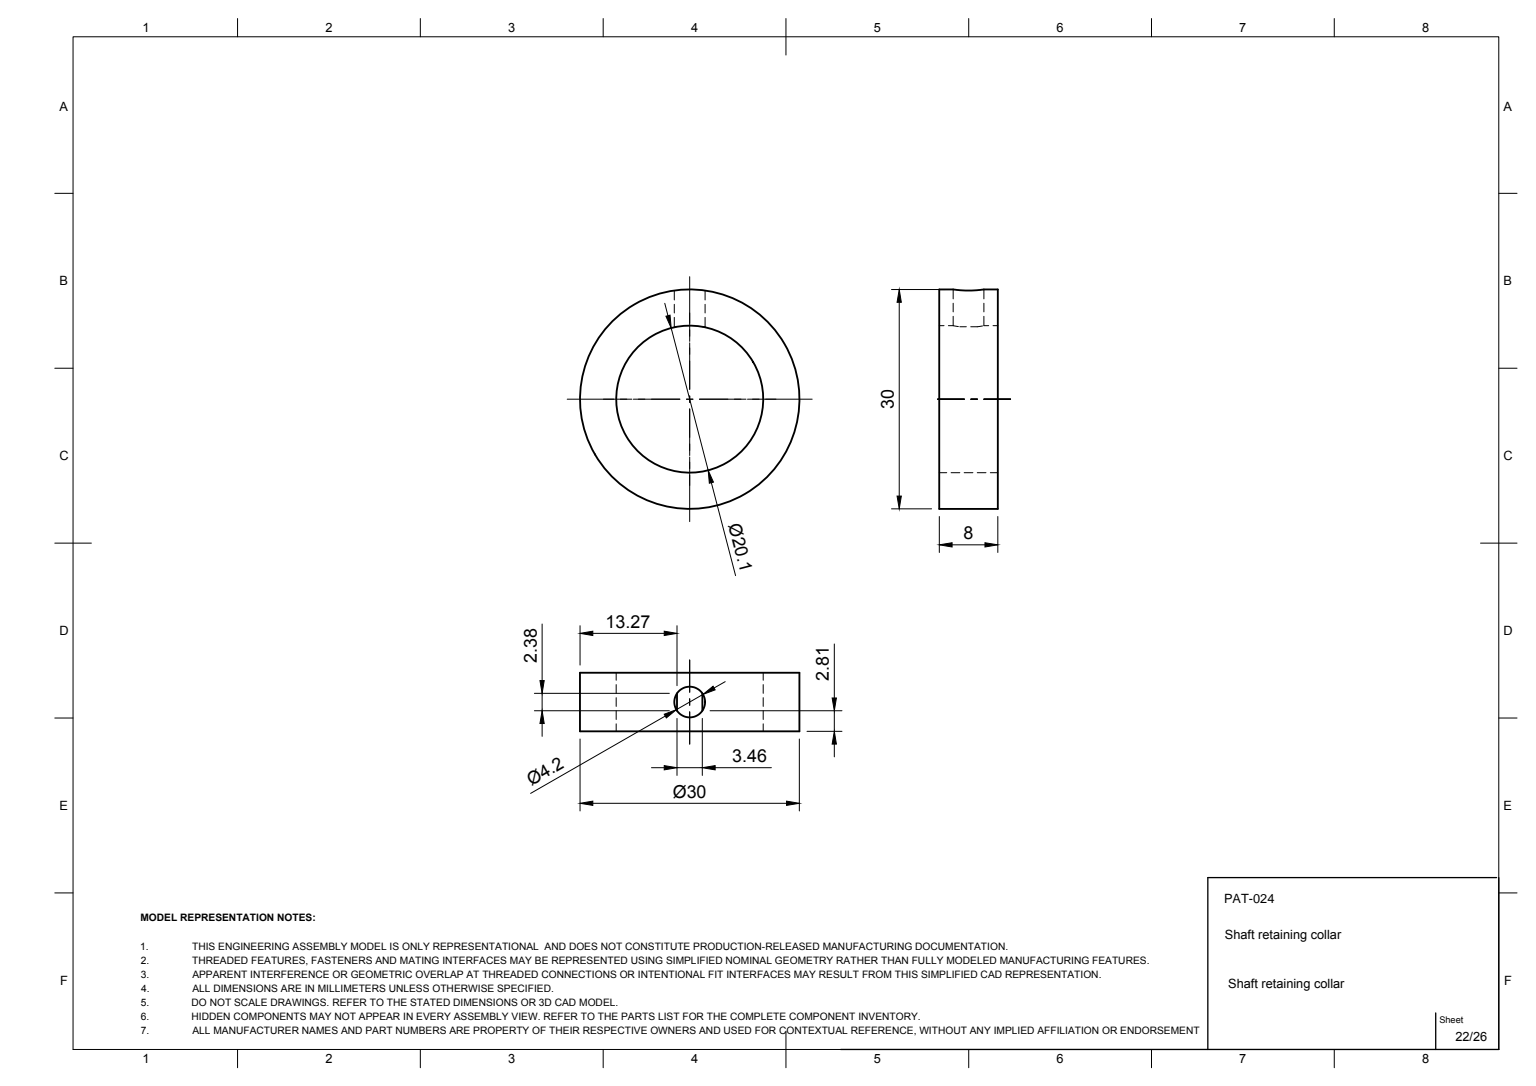
ISO-10303-21;
HEADER;
/* Generated by software containing ST-Developer
 * from STEP Tools, Inc. (www.steptools.com) 
 */

FILE_DESCRIPTION(
/* description */ ('Compact handwheel screw vise'),
/* implementation_level */ '2;1');

FILE_NAME(
/* name */ 'Shaft retaining collar.step',
/* time_stamp */ '2026-10-29T16:08:22-07:00',
/* author */ (''),
/* organization */ (''),
/* preprocessor_version */ 'ST-DEVELOPER v20.2',
/* originating_system */ 'Autodesk Translation Framework v15.17.0.0',
/* authorisation */ '');

FILE_SCHEMA (('AUTOMOTIVE_DESIGN { 1 0 10303 214 3 1 1 }'));
ENDSEC;

DATA;
#10=MECHANICAL_DESIGN_GEOMETRIC_PRESENTATION_REPRESENTATION('',(#672),#25074);
#531=B_SPLINE_CURVE_WITH_KNOTS('',3,(#24543,#24544,#24545,#24546,#24547,
#24548,#24549,#24550),.UNSPECIFIED.,.F.,.F.,(4,2,2,4),(0.756005737987019,
0.793568827564653,0.872922520054208,0.952276212543762),.UNSPECIFIED.);
#532=B_SPLINE_CURVE_WITH_KNOTS('',3,(#24553,#24554,#24555,#24556,#24557,
#24558,#24559,#24560,#24561,#24562,#24563,#24564,#24565,#24566),
 .UNSPECIFIED.,.F.,.F.,(4,2,2,2,2,2,4),(0.121154929624509,0.158718019202145,
0.238071711691699,0.317425404181254,0.396779096670809,0.476132789160363,
0.513695878738001),.UNSPECIFIED.);
#533=B_SPLINE_CURVE_WITH_KNOTS('',3,(#24567,#24568,#24569,#24570,#24571,
#24572,#24573,#24574),.UNSPECIFIED.,.F.,.F.,(4,2,2,4),(0.952276212543762,
1.03162990503332,1.11098359752287,1.14854668710052),.UNSPECIFIED.);
#534=B_SPLINE_CURVE_WITH_KNOTS('',3,(#24578,#24579,#24580,#24581,#24582,
#24583,#24584,#24585,#24586,#24587),.UNSPECIFIED.,.F.,.F.,(4,2,2,2,4),(0.,
0.0792165807733642,0.158433161546728,0.237648697074572,0.316864232602417),
 .UNSPECIFIED.);
#535=B_SPLINE_CURVE_WITH_KNOTS('',3,(#24588,#24589,#24590,#24591,#24592,
#24593,#24594,#24595,#24596,#24597,#24598,#24599,#24600,#24601,#24602,#24603,
#24604,#24605,#24606,#24607,#24608,#24609,#24610,#24611,#24612,#24613),
 .UNSPECIFIED.,.F.,.F.,(4,2,2,2,2,2,2,2,2,2,2,2,4),(0.316864232602417,0.396079768130261,
0.475295303658105,0.554511884431469,0.633728465204833,0.712945045978197,
0.792161626751562,0.871377162279406,0.95059269780725,1.02980823333509,1.10902376886294,
1.1882403496363,1.26745693040967),.UNSPECIFIED.);
#608=SHAPE_REPRESENTATION_RELATIONSHIP('SRR','None',#25219,#636);
#636=ADVANCED_BREP_SHAPE_REPRESENTATION('',(#705),#25066);
#672=STYLED_ITEM('',(#25439),#705);
#705=MANIFOLD_SOLID_BREP('Body1',#8083);
#804=FACE_BOUND('',#1977,.T.);
#805=FACE_BOUND('',#1979,.T.);
#806=FACE_BOUND('',#1981,.T.);
#807=FACE_BOUND('',#1983,.T.);
#964=PLANE('',#9053);
#965=PLANE('',#9057);
#966=PLANE('',#9064);
#967=PLANE('',#9065);
#1411=FACE_OUTER_BOUND('',#1973,.T.);
#1412=FACE_OUTER_BOUND('',#1974,.T.);
#1413=FACE_OUTER_BOUND('',#1975,.T.);
#1414=FACE_OUTER_BOUND('',#1976,.T.);
#1415=FACE_OUTER_BOUND('',#1978,.T.);
#1416=FACE_OUTER_BOUND('',#1980,.T.);
#1417=FACE_OUTER_BOUND('',#1982,.T.);
#1973=EDGE_LOOP('',(#7047,#7048));
#1974=EDGE_LOOP('',(#7049,#7050,#7051,#7052,#7053,#7054,#7055,#7056,#7057));
#1975=EDGE_LOOP('',(#7058,#7059));
#1976=EDGE_LOOP('',(#7060,#7061,#7062,#7063));
#1977=EDGE_LOOP('',(#7064,#7065,#7066,#7067,#7068));
#1978=EDGE_LOOP('',(#7069,#7070,#7071,#7072));
#1979=EDGE_LOOP('',(#7073,#7074));
#1980=EDGE_LOOP('',(#7075));
#1981=EDGE_LOOP('',(#7076));
#1982=EDGE_LOOP('',(#7077));
#1983=EDGE_LOOP('',(#7078));
#2471=LINE('',#24538,#2979);
#2472=LINE('',#24576,#2980);
#2473=LINE('',#24615,#2981);
#2474=LINE('',#24620,#2982);
#2475=LINE('',#24626,#2983);
#2979=VECTOR('',#10919,1.);
#2980=VECTOR('',#10926,0.210000000000001);
#2981=VECTOR('',#10929,1.);
#2982=VECTOR('',#10934,1.005);
#2983=VECTOR('',#10941,1.5);
#3293=CIRCLE('',#9054,0.210000000000001);
#3294=CIRCLE('',#9056,0.210000000000001);
#3295=CIRCLE('',#9059,1.005);
#3296=CIRCLE('',#9060,1.005);
#3297=CIRCLE('',#9062,1.5);
#3298=CIRCLE('',#9063,1.5);
#3968=VERTEX_POINT('',#24536);
#3969=VERTEX_POINT('',#24537);
#3970=VERTEX_POINT('',#24541);
#3971=VERTEX_POINT('',#24542);
#3972=VERTEX_POINT('',#24551);
#3973=VERTEX_POINT('',#24575);
#3974=VERTEX_POINT('',#24577);
#3975=VERTEX_POINT('',#24617);
#3976=VERTEX_POINT('',#24619);
#3977=VERTEX_POINT('',#24623);
#3978=VERTEX_POINT('',#24625);
#5010=EDGE_CURVE('',#3968,#3969,#2471,.T.);
#5011=EDGE_CURVE('',#3968,#3969,#3293,.T.);
#5012=EDGE_CURVE('',#3970,#3971,#531,.T.);
#5013=EDGE_CURVE('',#3972,#3970,#3294,.T.);
#5014=EDGE_CURVE('',#3969,#3972,#532,.T.);
#5015=EDGE_CURVE('',#3971,#3968,#533,.T.);
#5016=EDGE_CURVE('',#3971,#3973,#2472,.T.);
#5017=EDGE_CURVE('',#3974,#3973,#534,.T.);
#5018=EDGE_CURVE('',#3973,#3974,#535,.T.);
#5019=EDGE_CURVE('',#3972,#3970,#2473,.T.);
#5020=EDGE_CURVE('',#3975,#3975,#3295,.T.);
#5021=EDGE_CURVE('',#3975,#3976,#2474,.T.);
#5022=EDGE_CURVE('',#3976,#3976,#3296,.T.);
#5023=EDGE_CURVE('',#3977,#3977,#3297,.T.);
#5024=EDGE_CURVE('',#3977,#3978,#2475,.T.);
#5025=EDGE_CURVE('',#3978,#3978,#3298,.T.);
#7047=ORIENTED_EDGE('',*,*,#5010,.F.);
#7048=ORIENTED_EDGE('',*,*,#5011,.T.);
#7049=ORIENTED_EDGE('',*,*,#5012,.F.);
#7050=ORIENTED_EDGE('',*,*,#5013,.F.);
#7051=ORIENTED_EDGE('',*,*,#5014,.F.);
#7052=ORIENTED_EDGE('',*,*,#5011,.F.);
#7053=ORIENTED_EDGE('',*,*,#5015,.F.);
#7054=ORIENTED_EDGE('',*,*,#5016,.T.);
#7055=ORIENTED_EDGE('',*,*,#5017,.F.);
#7056=ORIENTED_EDGE('',*,*,#5018,.F.);
#7057=ORIENTED_EDGE('',*,*,#5016,.F.);
#7058=ORIENTED_EDGE('',*,*,#5019,.F.);
#7059=ORIENTED_EDGE('',*,*,#5013,.T.);
#7060=ORIENTED_EDGE('',*,*,#5020,.F.);
#7061=ORIENTED_EDGE('',*,*,#5021,.T.);
#7062=ORIENTED_EDGE('',*,*,#5022,.T.);
#7063=ORIENTED_EDGE('',*,*,#5021,.F.);
#7064=ORIENTED_EDGE('',*,*,#5014,.T.);
#7065=ORIENTED_EDGE('',*,*,#5019,.T.);
#7066=ORIENTED_EDGE('',*,*,#5012,.T.);
#7067=ORIENTED_EDGE('',*,*,#5015,.T.);
#7068=ORIENTED_EDGE('',*,*,#5010,.T.);
#7069=ORIENTED_EDGE('',*,*,#5023,.F.);
#7070=ORIENTED_EDGE('',*,*,#5024,.T.);
#7071=ORIENTED_EDGE('',*,*,#5025,.T.);
#7072=ORIENTED_EDGE('',*,*,#5024,.F.);
#7073=ORIENTED_EDGE('',*,*,#5017,.T.);
#7074=ORIENTED_EDGE('',*,*,#5018,.T.);
#7075=ORIENTED_EDGE('',*,*,#5023,.T.);
#7076=ORIENTED_EDGE('',*,*,#5020,.T.);
#7077=ORIENTED_EDGE('',*,*,#5025,.F.);
#7078=ORIENTED_EDGE('',*,*,#5022,.F.);
#7565=CYLINDRICAL_SURFACE('',#9055,0.210000000000001);
#7566=CYLINDRICAL_SURFACE('',#9058,1.005);
#7567=CYLINDRICAL_SURFACE('',#9061,1.5);
#7981=ADVANCED_FACE('',(#1411),#964,.T.);
#7982=ADVANCED_FACE('',(#1412),#7565,.F.);
#7983=ADVANCED_FACE('',(#1413),#965,.T.);
#7984=ADVANCED_FACE('',(#1414,#804),#7566,.F.);
#7985=ADVANCED_FACE('',(#1415,#805),#7567,.T.);
#7986=ADVANCED_FACE('',(#1416,#806),#966,.T.);
#7987=ADVANCED_FACE('',(#1417,#807),#967,.F.);
#8083=CLOSED_SHELL('',(#7981,#7982,#7983,#7984,#7985,#7986,#7987));
#9052=AXIS2_PLACEMENT_3D('',#24534,#10915,#10916);
#9053=AXIS2_PLACEMENT_3D('',#24535,#10917,#10918);
#9054=AXIS2_PLACEMENT_3D('',#24539,#10920,#10921);
#9055=AXIS2_PLACEMENT_3D('',#24540,#10922,#10923);
#9056=AXIS2_PLACEMENT_3D('',#24552,#10924,#10925);
#9057=AXIS2_PLACEMENT_3D('',#24614,#10927,#10928);
#9058=AXIS2_PLACEMENT_3D('',#24616,#10930,#10931);
#9059=AXIS2_PLACEMENT_3D('',#24618,#10932,#10933);
#9060=AXIS2_PLACEMENT_3D('',#24621,#10935,#10936);
#9061=AXIS2_PLACEMENT_3D('',#24622,#10937,#10938);
#9062=AXIS2_PLACEMENT_3D('',#24624,#10939,#10940);
#9063=AXIS2_PLACEMENT_3D('',#24627,#10942,#10943);
#9064=AXIS2_PLACEMENT_3D('',#24628,#10944,#10945);
#9065=AXIS2_PLACEMENT_3D('',#24629,#10946,#10947);
#10915=DIRECTION('axis',(0.,0.,1.));
#10916=DIRECTION('refdir',(1.,0.,0.));
#10917=DIRECTION('center_axis',(0.,1.,0.));
#10918=DIRECTION('ref_axis',(1.,0.,0.));
#10919=DIRECTION('',(1.,0.,0.));
#10920=DIRECTION('center_axis',(0.,1.,0.));
#10921=DIRECTION('ref_axis',(1.,0.,0.));
#10922=DIRECTION('center_axis',(0.,1.,0.));
#10923=DIRECTION('ref_axis',(1.,0.,0.));
#10924=DIRECTION('center_axis',(0.,1.,0.));
#10925=DIRECTION('ref_axis',(1.,0.,0.));
#10926=DIRECTION('',(0.,1.,0.));
#10927=DIRECTION('center_axis',(0.,1.,0.));
#10928=DIRECTION('ref_axis',(1.,0.,0.));
#10929=DIRECTION('',(-1.,0.,0.));
#10930=DIRECTION('center_axis',(1.,0.,0.));
#10931=DIRECTION('ref_axis',(0.,0.,-1.));
#10932=DIRECTION('center_axis',(-1.,0.,0.));
#10933=DIRECTION('ref_axis',(0.,0.,-1.));
#10934=DIRECTION('',(-1.,0.,0.));
#10935=DIRECTION('center_axis',(-1.,0.,0.));
#10936=DIRECTION('ref_axis',(0.,0.,-1.));
#10937=DIRECTION('center_axis',(1.,0.,0.));
#10938=DIRECTION('ref_axis',(0.,0.,-1.));
#10939=DIRECTION('center_axis',(1.,0.,0.));
#10940=DIRECTION('ref_axis',(0.,0.,-1.));
#10941=DIRECTION('',(-1.,0.,0.));
#10942=DIRECTION('center_axis',(1.,0.,0.));
#10943=DIRECTION('ref_axis',(0.,0.,-1.));
#10944=DIRECTION('center_axis',(1.,0.,0.));
#10945=DIRECTION('ref_axis',(0.,0.,-1.));
#10946=DIRECTION('center_axis',(1.,0.,0.));
#10947=DIRECTION('ref_axis',(0.,0.,-1.));
#24534=CARTESIAN_POINT('',(0.,0.,0.));
#24535=CARTESIAN_POINT('Origin',(25.8,0.99,4.));
#24536=CARTESIAN_POINT('',(25.6809411910021,0.99,4.17298843892006));
#24537=CARTESIAN_POINT('',(25.9190588089979,0.99,4.17298843892006));
#24538=CARTESIAN_POINT('',(25.4,0.99,4.17298843892006));
#24539=CARTESIAN_POINT('Origin',(25.8,0.99,4.));
#24540=CARTESIAN_POINT('Origin',(25.8,0.99,4.));
#24541=CARTESIAN_POINT('',(25.6809411910021,0.99,3.82701156107994));
#24542=CARTESIAN_POINT('',(25.59,1.005,4.));
#24543=CARTESIAN_POINT('Ctrl Pts',(25.6809411910021,0.989999999999999,3.82701156107994));
#24544=CARTESIAN_POINT('Ctrl Pts',(25.6701985776047,0.99129192197638,3.83440513468868));
#24545=CARTESIAN_POINT('Ctrl Pts',(25.6603122906273,0.992653949439047,3.84270286127439));
#24546=CARTESIAN_POINT('Ctrl Pts',(25.6329072257467,0.996748084390898,3.87010792615492));
#24547=CARTESIAN_POINT('Ctrl Pts',(25.6167579436671,0.999695893276376,3.89366983224072));
#24548=CARTESIAN_POINT('Ctrl Pts',(25.5953022060351,1.00385029472357,3.94538709536759));
#24549=CARTESIAN_POINT('Ctrl Pts',(25.59,1.005,3.97354876917015));
#24550=CARTESIAN_POINT('Ctrl Pts',(25.59,1.005,4.));
#24551=CARTESIAN_POINT('',(25.9190588089979,0.99,3.82701156107994));
#24552=CARTESIAN_POINT('Origin',(25.8,0.99,4.));
#24553=CARTESIAN_POINT('Ctrl Pts',(25.9190588089979,0.99,4.17298843892006));
#24554=CARTESIAN_POINT('Ctrl Pts',(25.9298014223953,0.991291921976381,4.16559486531132));
#24555=CARTESIAN_POINT('Ctrl Pts',(25.9396877093727,0.992653949439047,4.15729713872561));
#24556=CARTESIAN_POINT('Ctrl Pts',(25.9670927742533,0.996748084390898,4.12989207384508));
#24557=CARTESIAN_POINT('Ctrl Pts',(25.9832420563329,0.999695893276376,4.10633016775929));
#24558=CARTESIAN_POINT('Ctrl Pts',(26.0046977939649,1.00385029472357,4.05461290463241));
#24559=CARTESIAN_POINT('Ctrl Pts',(26.01,1.005,4.02645123082985));
#24560=CARTESIAN_POINT('Ctrl Pts',(26.01,1.005,3.97354876917015));
#24561=CARTESIAN_POINT('Ctrl Pts',(26.0046977939649,1.00385029472357,3.94538709536759));
#24562=CARTESIAN_POINT('Ctrl Pts',(25.9832420563329,0.999695893276376,3.89366983224072));
#24563=CARTESIAN_POINT('Ctrl Pts',(25.9670927742533,0.996748084390898,3.87010792615492));
#24564=CARTESIAN_POINT('Ctrl Pts',(25.9396877093727,0.992653949439047,3.84270286127439));
#24565=CARTESIAN_POINT('Ctrl Pts',(25.9298014223953,0.991291921976381,3.83440513468868));
#24566=CARTESIAN_POINT('Ctrl Pts',(25.9190588089979,0.99,3.82701156107994));
#24567=CARTESIAN_POINT('Ctrl Pts',(25.59,1.005,4.));
#24568=CARTESIAN_POINT('Ctrl Pts',(25.59,1.005,4.02645123082985));
#24569=CARTESIAN_POINT('Ctrl Pts',(25.5953022060351,1.00385029472357,4.05461290463241));
#24570=CARTESIAN_POINT('Ctrl Pts',(25.6167579436671,0.999695893276376,4.10633016775929));
#24571=CARTESIAN_POINT('Ctrl Pts',(25.6329072257467,0.996748084390898,4.12989207384508));
#24572=CARTESIAN_POINT('Ctrl Pts',(25.6603122906273,0.992653949439047,4.15729713872561));
#24573=CARTESIAN_POINT('Ctrl Pts',(25.6701985776047,0.991291921976381,4.16559486531132));
#24574=CARTESIAN_POINT('Ctrl Pts',(25.6809411910021,0.99,4.17298843892006));
#24575=CARTESIAN_POINT('',(25.59,1.5,4.));
#24576=CARTESIAN_POINT('',(25.59,0.99,4.));
#24577=CARTESIAN_POINT('',(25.8,1.48522725533839,4.21));
#24578=CARTESIAN_POINT('Ctrl Pts',(25.8,1.48522725533839,4.21));
#24579=CARTESIAN_POINT('Ctrl Pts',(25.7735944730755,1.48522725533839,4.21));
#24580=CARTESIAN_POINT('Ctrl Pts',(25.7454529259093,1.48600415954412,4.2047157372696));
#24581=CARTESIAN_POINT('Ctrl Pts',(25.6937237310949,1.48880073282317,4.18327376303633));
#24582=CARTESIAN_POINT('Ctrl Pts',(25.670133075872,1.49077897157582,4.16711792397039));
#24583=CARTESIAN_POINT('Ctrl Pts',(25.632882321789,1.49448481141327,4.12986716988737));
#24584=CARTESIAN_POINT('Ctrl Pts',(25.6167262899986,1.49645455657129,4.10627640830577));
#24585=CARTESIAN_POINT('Ctrl Pts',(25.5952841751738,1.49923165515646,4.0545468514059));
#24586=CARTESIAN_POINT('Ctrl Pts',(25.59,1.5,4.02640517850928));
#24587=CARTESIAN_POINT('Ctrl Pts',(25.59,1.5,4.));
#24588=CARTESIAN_POINT('Ctrl Pts',(25.59,1.5,4.));
#24589=CARTESIAN_POINT('Ctrl Pts',(25.59,1.5,3.97359482149072));
#24590=CARTESIAN_POINT('Ctrl Pts',(25.5952841751738,1.49923165515646,3.9454531485941));
#24591=CARTESIAN_POINT('Ctrl Pts',(25.6167262899986,1.49645455657129,3.89372359169423));
#24592=CARTESIAN_POINT('Ctrl Pts',(25.632882321789,1.49448481141327,3.87013283011263));
#24593=CARTESIAN_POINT('Ctrl Pts',(25.670133075872,1.49077897157582,3.83288207602961));
#24594=CARTESIAN_POINT('Ctrl Pts',(25.6937237310949,1.48880073282317,3.81672623696366));
#24595=CARTESIAN_POINT('Ctrl Pts',(25.7454529259093,1.48600415954412,3.7952842627304));
#24596=CARTESIAN_POINT('Ctrl Pts',(25.7735944730755,1.48522725533839,3.79));
#24597=CARTESIAN_POINT('Ctrl Pts',(25.8264055269245,1.48522725533839,3.79));
#24598=CARTESIAN_POINT('Ctrl Pts',(25.8545470740907,1.48600415954412,3.7952842627304));
#24599=CARTESIAN_POINT('Ctrl Pts',(25.9062762689051,1.48880073282317,3.81672623696367));
#24600=CARTESIAN_POINT('Ctrl Pts',(25.929866924128,1.49077897157582,3.83288207602961));
#24601=CARTESIAN_POINT('Ctrl Pts',(25.967117678211,1.49448481141327,3.87013283011263));
#24602=CARTESIAN_POINT('Ctrl Pts',(25.9832737100014,1.49645455657129,3.89372359169423));
#24603=CARTESIAN_POINT('Ctrl Pts',(26.0047158248262,1.49923165515646,3.9454531485941));
#24604=CARTESIAN_POINT('Ctrl Pts',(26.01,1.5,3.97359482149072));
#24605=CARTESIAN_POINT('Ctrl Pts',(26.01,1.5,4.02640517850928));
#24606=CARTESIAN_POINT('Ctrl Pts',(26.0047158248262,1.49923165515646,4.0545468514059));
#24607=CARTESIAN_POINT('Ctrl Pts',(25.9832737100014,1.49645455657129,4.10627640830577));
#24608=CARTESIAN_POINT('Ctrl Pts',(25.967117678211,1.49448481141327,4.12986716988737));
#24609=CARTESIAN_POINT('Ctrl Pts',(25.929866924128,1.49077897157582,4.16711792397039));
#24610=CARTESIAN_POINT('Ctrl Pts',(25.9062762689051,1.48880073282317,4.18327376303633));
#24611=CARTESIAN_POINT('Ctrl Pts',(25.8545470740907,1.48600415954412,4.20471573726959));
#24612=CARTESIAN_POINT('Ctrl Pts',(25.8264055269245,1.48522725533839,4.21));
#24613=CARTESIAN_POINT('Ctrl Pts',(25.8,1.48522725533839,4.21));
#24614=CARTESIAN_POINT('Origin',(25.8,0.99,4.));
#24615=CARTESIAN_POINT('',(25.4,0.99,3.82701156107994));
#24616=CARTESIAN_POINT('Origin',(25.4,0.,4.));
#24617=CARTESIAN_POINT('',(26.2,-1.23077003314309E-16,5.005));
#24618=CARTESIAN_POINT('Origin',(26.2,0.,4.));
#24619=CARTESIAN_POINT('',(25.4,-1.23077003314309E-16,5.005));
#24620=CARTESIAN_POINT('',(25.4,-1.23077003314309E-16,5.005));
#24621=CARTESIAN_POINT('Origin',(25.4,0.,4.));
#24622=CARTESIAN_POINT('Origin',(25.4,0.,4.));
#24623=CARTESIAN_POINT('',(26.2,-1.83697019872103E-16,5.5));
#24624=CARTESIAN_POINT('Origin',(26.2,0.,4.));
#24625=CARTESIAN_POINT('',(25.4,-1.83697019872103E-16,5.5));
#24626=CARTESIAN_POINT('',(25.4,-1.83697019872103E-16,5.5));
#24627=CARTESIAN_POINT('Origin',(25.4,0.,4.));
#24628=CARTESIAN_POINT('Origin',(26.2,0.,4.));
#24629=CARTESIAN_POINT('Origin',(25.4,0.,4.));
#25032=UNCERTAINTY_MEASURE_WITH_UNIT(LENGTH_MEASURE(0.001),#25075,
'DISTANCE_ACCURACY_VALUE',
'Maximum model space distance between geometric entities at asserted c
onnectivities');
#25040=UNCERTAINTY_MEASURE_WITH_UNIT(LENGTH_MEASURE(0.001),#25075,
'DISTANCE_ACCURACY_VALUE',
'Maximum model space distance between geometric entities at asserted c
onnectivities');
#25066=(
GEOMETRIC_REPRESENTATION_CONTEXT(3)
GLOBAL_UNCERTAINTY_ASSIGNED_CONTEXT((#25032))
GLOBAL_UNIT_ASSIGNED_CONTEXT((#25075,#25077,#25078))
REPRESENTATION_CONTEXT('','3D')
);
#25074=(
GEOMETRIC_REPRESENTATION_CONTEXT(3)
GLOBAL_UNCERTAINTY_ASSIGNED_CONTEXT((#25040))
GLOBAL_UNIT_ASSIGNED_CONTEXT((#25075,#25077,#25078))
REPRESENTATION_CONTEXT('','3D')
);
#25075=(
LENGTH_UNIT()
NAMED_UNIT(*)
SI_UNIT(.CENTI.,.METRE.)
);
#25077=(
NAMED_UNIT(*)
PLANE_ANGLE_UNIT()
SI_UNIT($,.RADIAN.)
);
#25078=(
NAMED_UNIT(*)
SI_UNIT($,.STERADIAN.)
SOLID_ANGLE_UNIT()
);
#25104=SHAPE_DEFINITION_REPRESENTATION(#25153,#25219);
#25153=PRODUCT_DEFINITION_SHAPE('',$,#25253);
#25219=SHAPE_REPRESENTATION('',(#9052),#25066);
#25227=PRODUCT_DEFINITION_CONTEXT('part definition',#25328,'design');
#25253=PRODUCT_DEFINITION('Shaft retaining collar',
'Shaft retaining collar',#25286,#25227);
#25286=PRODUCT_DEFINITION_FORMATION('',$,#25355);
#25328=APPLICATION_CONTEXT(
'Core Data for Automotive Mechanical Design Process');
#25329=PRODUCT_CONTEXT('part definition',#25328,'mechanical');
#25355=PRODUCT('Shaft retaining collar','Shaft retaining collar',
'Shaft retaining collar',(#25329));
#25433=COLOUR_RGB('Grey',0.48,0.52,0.57);
#25434=FILL_AREA_STYLE_COLOUR('',#25433);
#25435=FILL_AREA_STYLE('',(#25434));
#25436=SURFACE_STYLE_FILL_AREA(#25435);
#25437=SURFACE_SIDE_STYLE('',(#25436));
#25438=SURFACE_STYLE_USAGE(.BOTH.,#25437);
#25439=PRESENTATION_STYLE_ASSIGNMENT((#25438));
ENDSEC;
END-ISO-10303-21;
